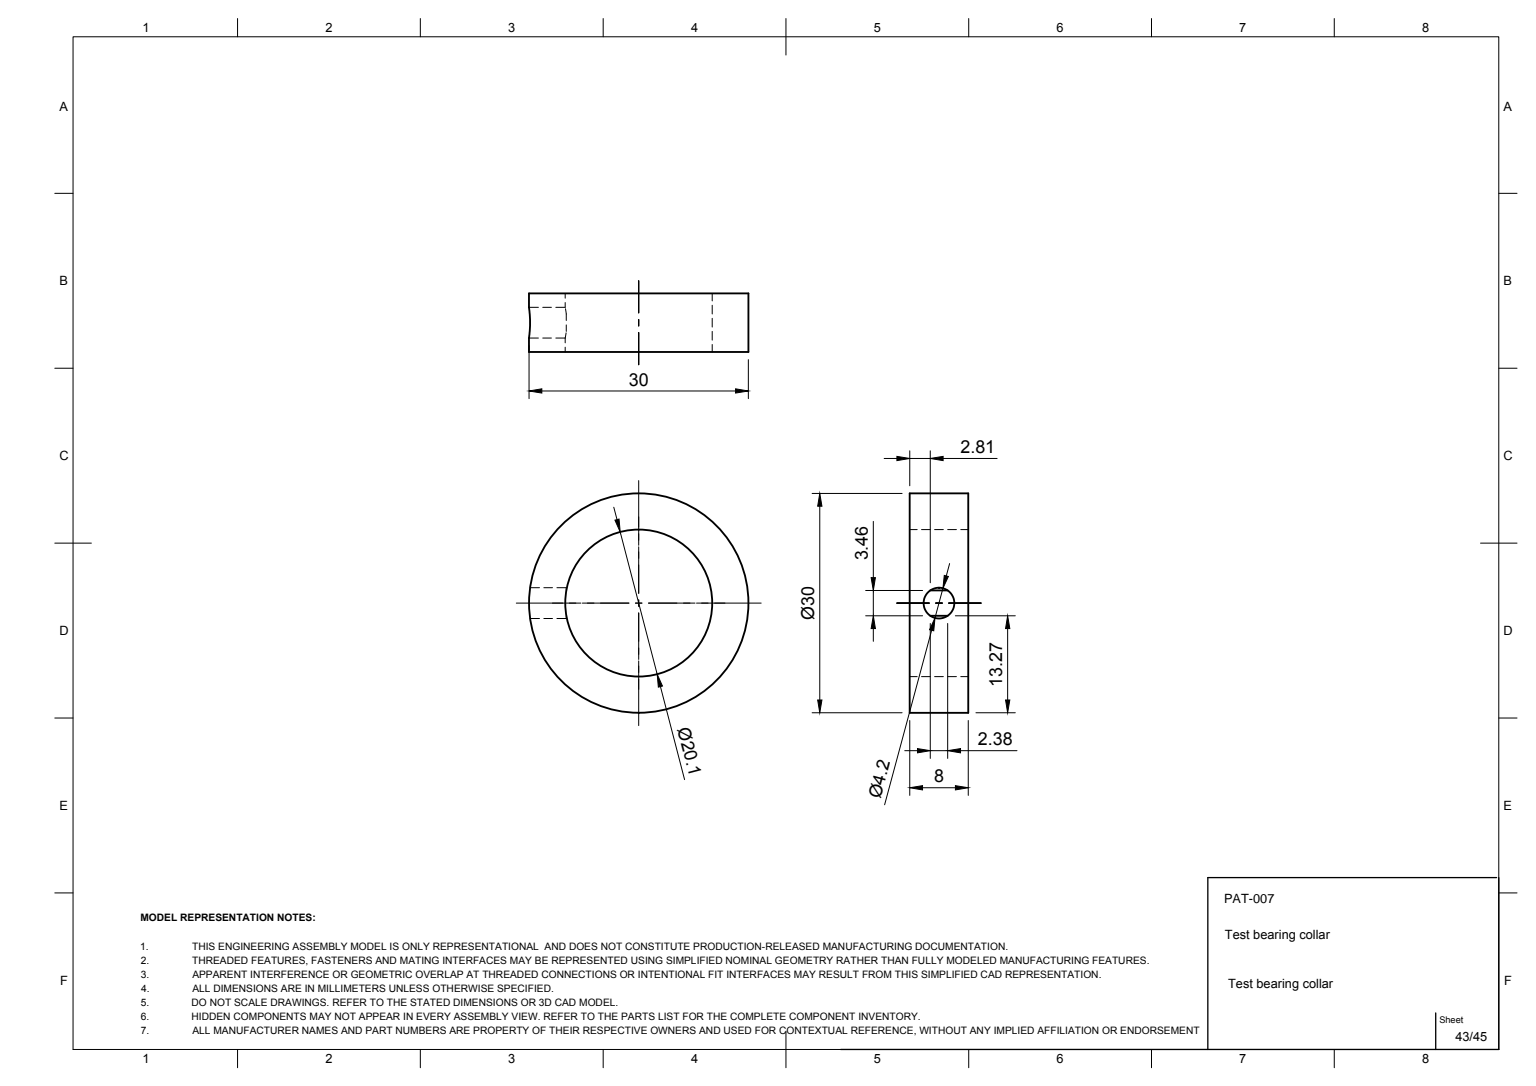
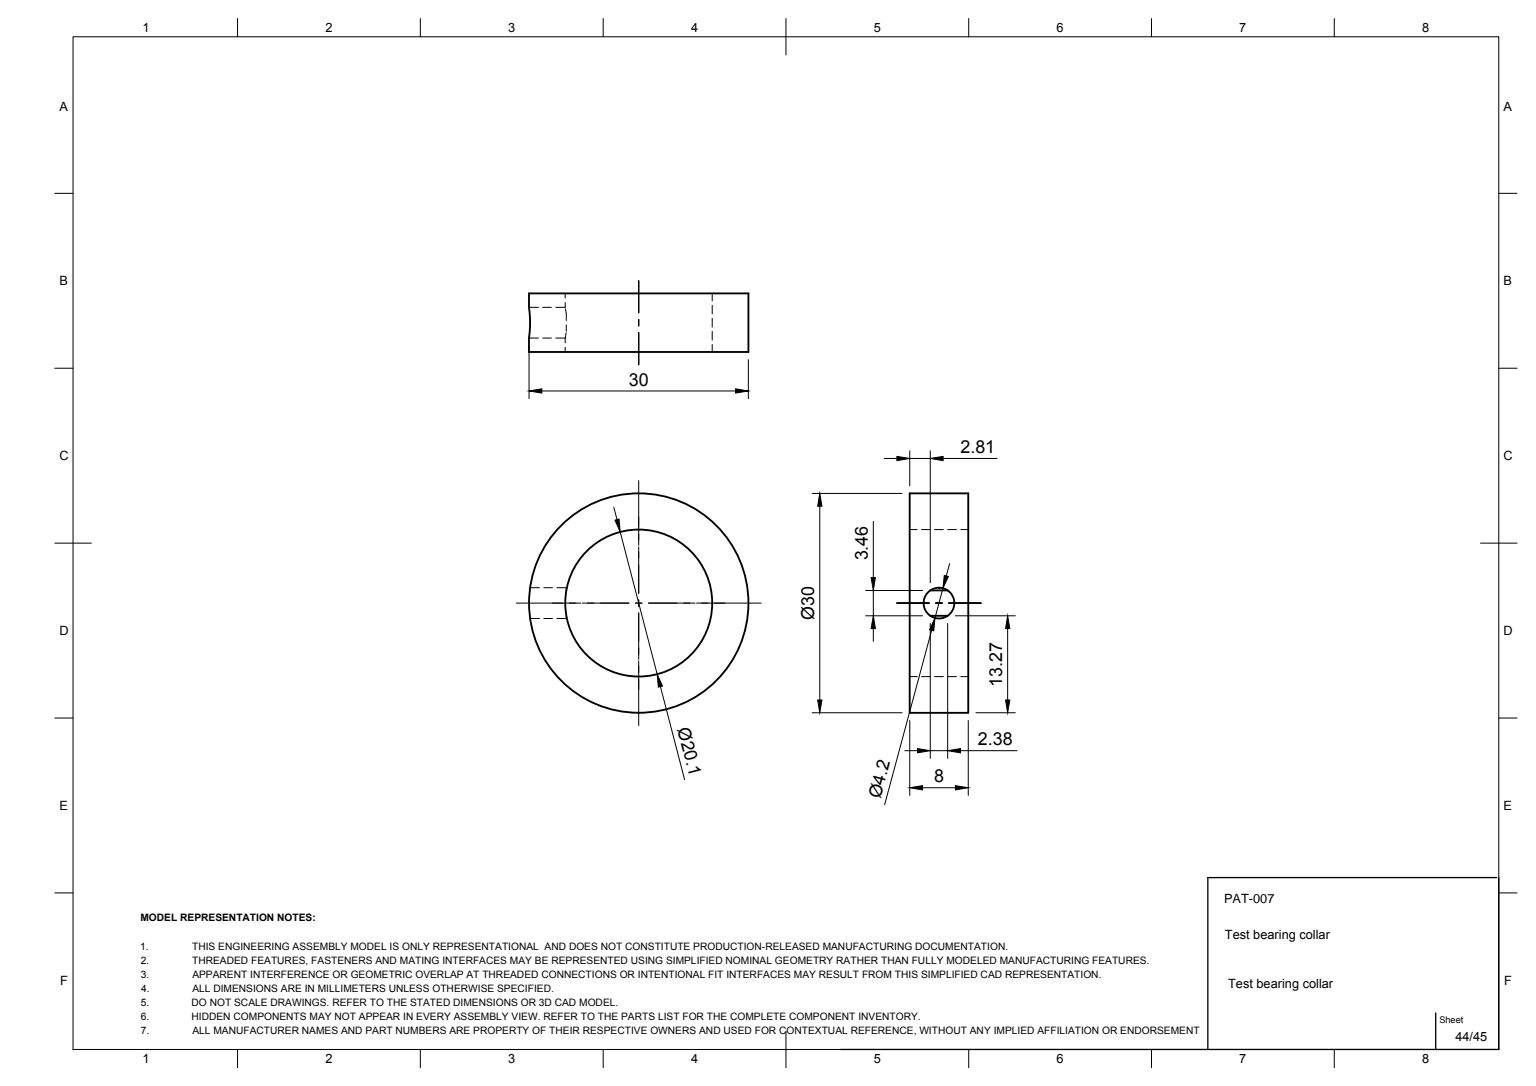
ISO-10303-21;
HEADER;
/* Generated by software containing ST-Developer
 * from STEP Tools, Inc. (www.steptools.com) 
 */

FILE_DESCRIPTION(
/* description */ ('Bearing friction torque test rig'),
/* implementation_level */ '2;1');

FILE_NAME(
/* name */ 'Test bearing collar.step',
/* time_stamp */ '2026-10-28T03:24:04-07:00',
/* author */ (''),
/* organization */ (''),
/* preprocessor_version */ 'ST-DEVELOPER v20.2',
/* originating_system */ 'Autodesk Translation Framework v15.17.0.0',
/* authorisation */ '');

FILE_SCHEMA (('AUTOMOTIVE_DESIGN { 1 0 10303 214 3 1 1 }'));
ENDSEC;

DATA;
#10=MECHANICAL_DESIGN_GEOMETRIC_PRESENTATION_REPRESENTATION('',(#589),#14822);
#383=B_SPLINE_CURVE_WITH_KNOTS('',3,(#14362,#14363,#14364,#14365,#14366,
#14367,#14368,#14369,#14370,#14371,#14372,#14373,#14374,#14375),
 .UNSPECIFIED.,.F.,.F.,(4,2,2,2,2,2,4),(0.75600573798702,0.793568827564647,
0.872922520054202,0.952276212543757,1.03162990503331,1.11098359752287,1.14854668710049),
 .UNSPECIFIED.);
#384=B_SPLINE_CURVE_WITH_KNOTS('',3,(#14381,#14382,#14383,#14384,#14385,
#14386,#14387,#14388,#14389,#14390,#14391,#14392,#14393,#14394,#14395,#14396,
#14397,#14398),.UNSPECIFIED.,.F.,.F.,(4,2,2,2,2,2,2,2,4),(0.,0.079216580773363,
0.158433161546726,0.23764869707457,0.316864232602414,0.396079768130259,
0.475295303658103,0.554511884431466,0.633728465204829),.UNSPECIFIED.);
#385=B_SPLINE_CURVE_WITH_KNOTS('',3,(#14399,#14400,#14401,#14402,#14403,
#14404,#14405,#14406,#14407,#14408,#14409,#14410,#14411,#14412,#14413,#14414,
#14415,#14416),.UNSPECIFIED.,.F.,.F.,(4,2,2,2,2,2,2,2,4),(0.633728465204829,
0.712945045978192,0.792161626751555,0.871377162279399,0.950592697807243,
1.02980823333509,1.10902376886293,1.18824034963629,1.26745693040966),
 .UNSPECIFIED.);
#386=B_SPLINE_CURVE_WITH_KNOTS('',3,(#14419,#14420,#14421,#14422,#14423,
#14424,#14425,#14426,#14427,#14428,#14429,#14430,#14431,#14432),
 .UNSPECIFIED.,.F.,.F.,(4,2,2,2,2,2,4),(0.121154929624515,0.158718019202143,
0.238071711691697,0.317425404181252,0.396779096670807,0.476132789160362,
0.513695878737989),.UNSPECIFIED.);
#496=SHAPE_REPRESENTATION_RELATIONSHIP('SRR','None',#15038,#535);
#535=ADVANCED_BREP_SHAPE_REPRESENTATION('',(#640),#14818);
#589=STYLED_ITEM('',(#15284),#640);
#640=MANIFOLD_SOLID_BREP('Body1',#7708);
#852=FACE_BOUND('',#2162,.T.);
#853=FACE_BOUND('',#2164,.T.);
#854=FACE_BOUND('',#2166,.T.);
#855=FACE_BOUND('',#2168,.T.);
#1077=PLANE('',#9072);
#1078=PLANE('',#9077);
#1079=PLANE('',#9084);
#1080=PLANE('',#9085);
#1505=FACE_OUTER_BOUND('',#2158,.T.);
#1506=FACE_OUTER_BOUND('',#2159,.T.);
#1507=FACE_OUTER_BOUND('',#2160,.T.);
#1508=FACE_OUTER_BOUND('',#2161,.T.);
#1509=FACE_OUTER_BOUND('',#2163,.T.);
#1510=FACE_OUTER_BOUND('',#2165,.T.);
#1511=FACE_OUTER_BOUND('',#2167,.T.);
#2158=EDGE_LOOP('',(#6868,#6869));
#2159=EDGE_LOOP('',(#6870,#6871,#6872,#6873,#6874,#6875,#6876,#6877,#6878));
#2160=EDGE_LOOP('',(#6879,#6880,#6881));
#2161=EDGE_LOOP('',(#6882,#6883,#6884,#6885));
#2162=EDGE_LOOP('',(#6886,#6887,#6888,#6889));
#2163=EDGE_LOOP('',(#6890,#6891,#6892,#6893));
#2164=EDGE_LOOP('',(#6894,#6895));
#2165=EDGE_LOOP('',(#6896));
#2166=EDGE_LOOP('',(#6897));
#2167=EDGE_LOOP('',(#6898));
#2168=EDGE_LOOP('',(#6899));
#2622=LINE('',#14358,#3066);
#2623=LINE('',#14379,#3067);
#2624=LINE('',#14434,#3068);
#2625=LINE('',#14439,#3069);
#2626=LINE('',#14445,#3070);
#3066=VECTOR('',#11431,1.);
#3067=VECTOR('',#11438,0.21);
#3068=VECTOR('',#11443,1.);
#3069=VECTOR('',#11448,1.005);
#3070=VECTOR('',#11455,1.5);
#3518=CIRCLE('',#9073,0.21);
#3519=CIRCLE('',#9075,0.21);
#3520=CIRCLE('',#9076,0.21);
#3521=CIRCLE('',#9079,1.005);
#3522=CIRCLE('',#9080,1.005);
#3523=CIRCLE('',#9082,1.5);
#3524=CIRCLE('',#9083,1.5);
#4141=VERTEX_POINT('',#14356);
#4142=VERTEX_POINT('',#14357);
#4143=VERTEX_POINT('',#14361);
#4144=VERTEX_POINT('',#14376);
#4145=VERTEX_POINT('',#14378);
#4146=VERTEX_POINT('',#14380);
#4147=VERTEX_POINT('',#14417);
#4148=VERTEX_POINT('',#14436);
#4149=VERTEX_POINT('',#14438);
#4150=VERTEX_POINT('',#14442);
#4151=VERTEX_POINT('',#14444);
#5060=EDGE_CURVE('',#4141,#4142,#2622,.T.);
#5061=EDGE_CURVE('',#4141,#4142,#3518,.T.);
#5062=EDGE_CURVE('',#4143,#4141,#383,.T.);
#5063=EDGE_CURVE('',#4144,#4143,#3519,.T.);
#5064=EDGE_CURVE('',#4144,#4145,#2623,.T.);
#5065=EDGE_CURVE('',#4146,#4145,#384,.T.);
#5066=EDGE_CURVE('',#4145,#4146,#385,.T.);
#5067=EDGE_CURVE('',#4147,#4144,#3520,.T.);
#5068=EDGE_CURVE('',#4142,#4147,#386,.T.);
#5069=EDGE_CURVE('',#4147,#4143,#2624,.T.);
#5070=EDGE_CURVE('',#4148,#4148,#3521,.T.);
#5071=EDGE_CURVE('',#4148,#4149,#2625,.T.);
#5072=EDGE_CURVE('',#4149,#4149,#3522,.T.);
#5073=EDGE_CURVE('',#4150,#4150,#3523,.T.);
#5074=EDGE_CURVE('',#4150,#4151,#2626,.T.);
#5075=EDGE_CURVE('',#4151,#4151,#3524,.T.);
#6868=ORIENTED_EDGE('',*,*,#5060,.F.);
#6869=ORIENTED_EDGE('',*,*,#5061,.T.);
#6870=ORIENTED_EDGE('',*,*,#5062,.F.);
#6871=ORIENTED_EDGE('',*,*,#5063,.F.);
#6872=ORIENTED_EDGE('',*,*,#5064,.T.);
#6873=ORIENTED_EDGE('',*,*,#5065,.F.);
#6874=ORIENTED_EDGE('',*,*,#5066,.F.);
#6875=ORIENTED_EDGE('',*,*,#5064,.F.);
#6876=ORIENTED_EDGE('',*,*,#5067,.F.);
#6877=ORIENTED_EDGE('',*,*,#5068,.F.);
#6878=ORIENTED_EDGE('',*,*,#5061,.F.);
#6879=ORIENTED_EDGE('',*,*,#5069,.F.);
#6880=ORIENTED_EDGE('',*,*,#5067,.T.);
#6881=ORIENTED_EDGE('',*,*,#5063,.T.);
#6882=ORIENTED_EDGE('',*,*,#5070,.F.);
#6883=ORIENTED_EDGE('',*,*,#5071,.T.);
#6884=ORIENTED_EDGE('',*,*,#5072,.T.);
#6885=ORIENTED_EDGE('',*,*,#5071,.F.);
#6886=ORIENTED_EDGE('',*,*,#5068,.T.);
#6887=ORIENTED_EDGE('',*,*,#5069,.T.);
#6888=ORIENTED_EDGE('',*,*,#5062,.T.);
#6889=ORIENTED_EDGE('',*,*,#5060,.T.);
#6890=ORIENTED_EDGE('',*,*,#5073,.F.);
#6891=ORIENTED_EDGE('',*,*,#5074,.T.);
#6892=ORIENTED_EDGE('',*,*,#5075,.T.);
#6893=ORIENTED_EDGE('',*,*,#5074,.F.);
#6894=ORIENTED_EDGE('',*,*,#5065,.T.);
#6895=ORIENTED_EDGE('',*,*,#5066,.T.);
#6896=ORIENTED_EDGE('',*,*,#5073,.T.);
#6897=ORIENTED_EDGE('',*,*,#5070,.T.);
#6898=ORIENTED_EDGE('',*,*,#5075,.F.);
#6899=ORIENTED_EDGE('',*,*,#5072,.F.);
#7195=CYLINDRICAL_SURFACE('',#9074,0.21);
#7196=CYLINDRICAL_SURFACE('',#9078,1.005);
#7197=CYLINDRICAL_SURFACE('',#9081,1.5);
#7616=ADVANCED_FACE('',(#1505),#1077,.T.);
#7617=ADVANCED_FACE('',(#1506),#7195,.F.);
#7618=ADVANCED_FACE('',(#1507),#1078,.T.);
#7619=ADVANCED_FACE('',(#1508,#852),#7196,.F.);
#7620=ADVANCED_FACE('',(#1509,#853),#7197,.T.);
#7621=ADVANCED_FACE('',(#1510,#854),#1079,.T.);
#7622=ADVANCED_FACE('',(#1511,#855),#1080,.F.);
#7708=CLOSED_SHELL('',(#7616,#7617,#7618,#7619,#7620,#7621,#7622));
#9071=AXIS2_PLACEMENT_3D('',#14354,#11427,#11428);
#9072=AXIS2_PLACEMENT_3D('',#14355,#11429,#11430);
#9073=AXIS2_PLACEMENT_3D('',#14359,#11432,#11433);
#9074=AXIS2_PLACEMENT_3D('',#14360,#11434,#11435);
#9075=AXIS2_PLACEMENT_3D('',#14377,#11436,#11437);
#9076=AXIS2_PLACEMENT_3D('',#14418,#11439,#11440);
#9077=AXIS2_PLACEMENT_3D('',#14433,#11441,#11442);
#9078=AXIS2_PLACEMENT_3D('',#14435,#11444,#11445);
#9079=AXIS2_PLACEMENT_3D('',#14437,#11446,#11447);
#9080=AXIS2_PLACEMENT_3D('',#14440,#11449,#11450);
#9081=AXIS2_PLACEMENT_3D('',#14441,#11451,#11452);
#9082=AXIS2_PLACEMENT_3D('',#14443,#11453,#11454);
#9083=AXIS2_PLACEMENT_3D('',#14446,#11456,#11457);
#9084=AXIS2_PLACEMENT_3D('',#14447,#11458,#11459);
#9085=AXIS2_PLACEMENT_3D('',#14448,#11460,#11461);
#11427=DIRECTION('axis',(0.,0.,1.));
#11428=DIRECTION('refdir',(1.,0.,0.));
#11429=DIRECTION('center_axis',(0.,0.,1.));
#11430=DIRECTION('ref_axis',(1.,0.,0.));
#11431=DIRECTION('',(0.,1.,0.));
#11432=DIRECTION('center_axis',(0.,0.,1.));
#11433=DIRECTION('ref_axis',(1.,0.,0.));
#11434=DIRECTION('center_axis',(0.,0.,1.));
#11435=DIRECTION('ref_axis',(1.,0.,0.));
#11436=DIRECTION('center_axis',(0.,0.,1.));
#11437=DIRECTION('ref_axis',(1.,0.,0.));
#11438=DIRECTION('',(0.,0.,1.));
#11439=DIRECTION('center_axis',(0.,0.,1.));
#11440=DIRECTION('ref_axis',(1.,0.,0.));
#11441=DIRECTION('center_axis',(0.,0.,1.));
#11442=DIRECTION('ref_axis',(1.,0.,0.));
#11443=DIRECTION('',(0.,-1.,0.));
#11444=DIRECTION('center_axis',(0.,1.,0.));
#11445=DIRECTION('ref_axis',(1.,0.,0.));
#11446=DIRECTION('center_axis',(0.,-1.,0.));
#11447=DIRECTION('ref_axis',(1.,0.,0.));
#11448=DIRECTION('',(0.,-1.,0.));
#11449=DIRECTION('center_axis',(0.,-1.,0.));
#11450=DIRECTION('ref_axis',(1.,0.,0.));
#11451=DIRECTION('center_axis',(0.,1.,0.));
#11452=DIRECTION('ref_axis',(1.,0.,0.));
#11453=DIRECTION('center_axis',(0.,1.,0.));
#11454=DIRECTION('ref_axis',(1.,0.,0.));
#11455=DIRECTION('',(0.,-1.,0.));
#11456=DIRECTION('center_axis',(0.,1.,0.));
#11457=DIRECTION('ref_axis',(1.,0.,0.));
#11458=DIRECTION('center_axis',(0.,1.,0.));
#11459=DIRECTION('ref_axis',(1.,0.,0.));
#11460=DIRECTION('center_axis',(0.,1.,0.));
#11461=DIRECTION('ref_axis',(1.,0.,0.));
#14354=CARTESIAN_POINT('',(0.,0.,0.));
#14355=CARTESIAN_POINT('Origin',(0.,-1.1,7.99));
#14356=CARTESIAN_POINT('',(0.172988438920056,-1.21905880899792,7.99));
#14357=CARTESIAN_POINT('',(0.172988438920056,-0.980941191002085,7.99));
#14358=CARTESIAN_POINT('',(0.172988438920056,-1.5,7.99));
#14359=CARTESIAN_POINT('Origin',(0.,-1.1,7.99));
#14360=CARTESIAN_POINT('Origin',(0.,-1.1,7.99));
#14361=CARTESIAN_POINT('',(-0.172988438920056,-1.21905880899792,7.99));
#14362=CARTESIAN_POINT('Ctrl Pts',(-0.172988438920056,-1.21905880899792,
7.99));
#14363=CARTESIAN_POINT('Ctrl Pts',(-0.165594865311315,-1.22980142239529,
7.99129192197638));
#14364=CARTESIAN_POINT('Ctrl Pts',(-0.157297138725606,-1.23968770937274,
7.99265394943905));
#14365=CARTESIAN_POINT('Ctrl Pts',(-0.129892073845076,-1.26709277425327,
7.9967480843909));
#14366=CARTESIAN_POINT('Ctrl Pts',(-0.106330167759285,-1.28324205633295,
7.99969589327638));
#14367=CARTESIAN_POINT('Ctrl Pts',(-0.0546129046324105,-1.30469779396491,
8.00385029472357));
#14368=CARTESIAN_POINT('Ctrl Pts',(-0.0264512308298516,-1.31,8.005));
#14369=CARTESIAN_POINT('Ctrl Pts',(0.0264512308298515,-1.31,8.005));
#14370=CARTESIAN_POINT('Ctrl Pts',(0.0546129046324104,-1.30469779396491,
8.00385029472357));
#14371=CARTESIAN_POINT('Ctrl Pts',(0.106330167759284,-1.28324205633295,
7.99969589327638));
#14372=CARTESIAN_POINT('Ctrl Pts',(0.129892073845076,-1.26709277425327,
7.9967480843909));
#14373=CARTESIAN_POINT('Ctrl Pts',(0.157297138725606,-1.23968770937274,
7.99265394943905));
#14374=CARTESIAN_POINT('Ctrl Pts',(0.165594865311314,-1.22980142239529,
7.99129192197638));
#14375=CARTESIAN_POINT('Ctrl Pts',(0.172988438920056,-1.21905880899792,
7.99));
#14376=CARTESIAN_POINT('',(-0.21,-1.1,7.99));
#14377=CARTESIAN_POINT('Origin',(0.,-1.1,7.99));
#14378=CARTESIAN_POINT('',(-0.21,-1.1,8.48522725533839));
#14379=CARTESIAN_POINT('',(-0.21,-1.1,7.99));
#14380=CARTESIAN_POINT('',(0.21,-1.1,8.48522725533839));
#14381=CARTESIAN_POINT('Ctrl Pts',(0.21,-1.1,8.48522725533839));
#14382=CARTESIAN_POINT('Ctrl Pts',(0.21,-1.12640552692445,8.48522725533839));
#14383=CARTESIAN_POINT('Ctrl Pts',(0.204715737269596,-1.15454707409071,
8.48600415954412));
#14384=CARTESIAN_POINT('Ctrl Pts',(0.183273763036331,-1.20627626890513,
8.48880073282317));
#14385=CARTESIAN_POINT('Ctrl Pts',(0.167117923970394,-1.22986692412796,
8.49077897157582));
#14386=CARTESIAN_POINT('Ctrl Pts',(0.129867169887369,-1.26711767821098,
8.49448481141327));
#14387=CARTESIAN_POINT('Ctrl Pts',(0.106276408305765,-1.28327371000135,
8.49645455657129));
#14388=CARTESIAN_POINT('Ctrl Pts',(0.0545468514059002,-1.30471582482622,
8.49923165515646));
#14389=CARTESIAN_POINT('Ctrl Pts',(0.0264051785092814,-1.31,8.5));
#14390=CARTESIAN_POINT('Ctrl Pts',(-0.0264051785092814,-1.31,8.5));
#14391=CARTESIAN_POINT('Ctrl Pts',(-0.0545468514059001,-1.30471582482622,
8.49923165515646));
#14392=CARTESIAN_POINT('Ctrl Pts',(-0.106276408305765,-1.28327371000135,
8.49645455657129));
#14393=CARTESIAN_POINT('Ctrl Pts',(-0.129867169887369,-1.26711767821098,
8.49448481141327));
#14394=CARTESIAN_POINT('Ctrl Pts',(-0.167117923970394,-1.22986692412796,
8.49077897157582));
#14395=CARTESIAN_POINT('Ctrl Pts',(-0.183273763036331,-1.20627626890513,
8.48880073282317));
#14396=CARTESIAN_POINT('Ctrl Pts',(-0.204715737269596,-1.15454707409071,
8.48600415954412));
#14397=CARTESIAN_POINT('Ctrl Pts',(-0.21,-1.12640552692445,8.48522725533839));
#14398=CARTESIAN_POINT('Ctrl Pts',(-0.21,-1.1,8.48522725533839));
#14399=CARTESIAN_POINT('Ctrl Pts',(-0.21,-1.1,8.48522725533839));
#14400=CARTESIAN_POINT('Ctrl Pts',(-0.21,-1.07359447307555,8.48522725533839));
#14401=CARTESIAN_POINT('Ctrl Pts',(-0.204715737269596,-1.04545292590929,
8.48600415954412));
#14402=CARTESIAN_POINT('Ctrl Pts',(-0.183273763036331,-0.993723731094873,
8.48880073282317));
#14403=CARTESIAN_POINT('Ctrl Pts',(-0.167117923970394,-0.970133075872044,
8.49077897157582));
#14404=CARTESIAN_POINT('Ctrl Pts',(-0.129867169887369,-0.932882321789019,
8.49448481141327));
#14405=CARTESIAN_POINT('Ctrl Pts',(-0.106276408305765,-0.916726289998648,
8.49645455657129));
#14406=CARTESIAN_POINT('Ctrl Pts',(-0.0545468514059001,-0.895284175173782,
8.49923165515646));
#14407=CARTESIAN_POINT('Ctrl Pts',(-0.0264051785092814,-0.89,8.5));
#14408=CARTESIAN_POINT('Ctrl Pts',(0.0264051785092814,-0.89,8.5));
#14409=CARTESIAN_POINT('Ctrl Pts',(0.0545468514059001,-0.895284175173782,
8.49923165515645));
#14410=CARTESIAN_POINT('Ctrl Pts',(0.106276408305765,-0.916726289998648,
8.49645455657129));
#14411=CARTESIAN_POINT('Ctrl Pts',(0.129867169887369,-0.932882321789019,
8.49448481141327));
#14412=CARTESIAN_POINT('Ctrl Pts',(0.167117923970394,-0.970133075872044,
8.49077897157582));
#14413=CARTESIAN_POINT('Ctrl Pts',(0.183273763036331,-0.993723731094873,
8.48880073282317));
#14414=CARTESIAN_POINT('Ctrl Pts',(0.204715737269596,-1.04545292590929,
8.48600415954412));
#14415=CARTESIAN_POINT('Ctrl Pts',(0.21,-1.07359447307555,8.48522725533839));
#14416=CARTESIAN_POINT('Ctrl Pts',(0.21,-1.1,8.48522725533839));
#14417=CARTESIAN_POINT('',(-0.172988438920056,-0.980941191002085,7.99));
#14418=CARTESIAN_POINT('Origin',(0.,-1.1,7.99));
#14419=CARTESIAN_POINT('Ctrl Pts',(0.172988438920056,-0.980941191002085,
7.99));
#14420=CARTESIAN_POINT('Ctrl Pts',(0.165594865311315,-0.970198577604708,
7.99129192197638));
#14421=CARTESIAN_POINT('Ctrl Pts',(0.157297138725606,-0.960312290627256,
7.99265394943905));
#14422=CARTESIAN_POINT('Ctrl Pts',(0.129892073845076,-0.932907225746726,
7.9967480843909));
#14423=CARTESIAN_POINT('Ctrl Pts',(0.106330167759284,-0.916757943667051,
7.99969589327638));
#14424=CARTESIAN_POINT('Ctrl Pts',(0.0546129046324105,-0.895302206035094,
8.00385029472357));
#14425=CARTESIAN_POINT('Ctrl Pts',(0.0264512308298516,-0.89,8.005));
#14426=CARTESIAN_POINT('Ctrl Pts',(-0.0264512308298516,-0.89,8.005));
#14427=CARTESIAN_POINT('Ctrl Pts',(-0.0546129046324105,-0.895302206035094,
8.00385029472357));
#14428=CARTESIAN_POINT('Ctrl Pts',(-0.106330167759284,-0.916757943667051,
7.99969589327638));
#14429=CARTESIAN_POINT('Ctrl Pts',(-0.129892073845076,-0.932907225746726,
7.9967480843909));
#14430=CARTESIAN_POINT('Ctrl Pts',(-0.157297138725606,-0.960312290627256,
7.99265394943905));
#14431=CARTESIAN_POINT('Ctrl Pts',(-0.165594865311314,-0.970198577604708,
7.99129192197638));
#14432=CARTESIAN_POINT('Ctrl Pts',(-0.172988438920056,-0.980941191002085,
7.99));
#14433=CARTESIAN_POINT('Origin',(0.,-1.1,7.99));
#14434=CARTESIAN_POINT('',(-0.172988438920056,-1.5,7.99));
#14435=CARTESIAN_POINT('Origin',(0.,-1.5,7.));
#14436=CARTESIAN_POINT('',(-1.005,-0.7,7.));
#14437=CARTESIAN_POINT('Origin',(0.,-0.7,7.));
#14438=CARTESIAN_POINT('',(-1.005,-1.5,7.));
#14439=CARTESIAN_POINT('',(-1.005,-1.5,7.));
#14440=CARTESIAN_POINT('Origin',(0.,-1.5,7.));
#14441=CARTESIAN_POINT('Origin',(0.,-1.5,7.));
#14442=CARTESIAN_POINT('',(-1.5,-0.7,7.));
#14443=CARTESIAN_POINT('Origin',(0.,-0.7,7.));
#14444=CARTESIAN_POINT('',(-1.5,-1.5,7.));
#14445=CARTESIAN_POINT('',(-1.5,-1.5,7.));
#14446=CARTESIAN_POINT('Origin',(0.,-1.5,7.));
#14447=CARTESIAN_POINT('Origin',(0.,-0.7,7.));
#14448=CARTESIAN_POINT('Origin',(0.,-1.5,7.));
#14773=UNCERTAINTY_MEASURE_WITH_UNIT(LENGTH_MEASURE(0.001),#14823,
'DISTANCE_ACCURACY_VALUE',
'Maximum model space distance between geometric entities at asserted c
onnectivities');
#14777=UNCERTAINTY_MEASURE_WITH_UNIT(LENGTH_MEASURE(0.001),#14823,
'DISTANCE_ACCURACY_VALUE',
'Maximum model space distance between geometric entities at asserted c
onnectivities');
#14818=(
GEOMETRIC_REPRESENTATION_CONTEXT(3)
GLOBAL_UNCERTAINTY_ASSIGNED_CONTEXT((#14773))
GLOBAL_UNIT_ASSIGNED_CONTEXT((#14823,#14825,#14826))
REPRESENTATION_CONTEXT('','3D')
);
#14822=(
GEOMETRIC_REPRESENTATION_CONTEXT(3)
GLOBAL_UNCERTAINTY_ASSIGNED_CONTEXT((#14777))
GLOBAL_UNIT_ASSIGNED_CONTEXT((#14823,#14825,#14826))
REPRESENTATION_CONTEXT('','3D')
);
#14823=(
LENGTH_UNIT()
NAMED_UNIT(*)
SI_UNIT(.CENTI.,.METRE.)
);
#14825=(
NAMED_UNIT(*)
PLANE_ANGLE_UNIT()
SI_UNIT($,.RADIAN.)
);
#14826=(
NAMED_UNIT(*)
SI_UNIT($,.STERADIAN.)
SOLID_ANGLE_UNIT()
);
#14867=SHAPE_DEFINITION_REPRESENTATION(#14977,#15038);
#14977=PRODUCT_DEFINITION_SHAPE('',$,#15083);
#15038=SHAPE_REPRESENTATION('',(#9071),#14818);
#15042=PRODUCT_DEFINITION_CONTEXT('part definition',#15176,'design');
#15083=PRODUCT_DEFINITION('Test bearing collar','Test bearing collar',#15127,
#15042);
#15127=PRODUCT_DEFINITION_FORMATION('',$,#15218);
#15176=APPLICATION_CONTEXT(
'Core Data for Automotive Mechanical Design Process');
#15177=PRODUCT_CONTEXT('part definition',#15176,'mechanical');
#15218=PRODUCT('Test bearing collar','Test bearing collar',
'Test bearing collar',(#15177));
#15278=COLOUR_RGB('Grey',0.48,0.52,0.57);
#15279=FILL_AREA_STYLE_COLOUR('',#15278);
#15280=FILL_AREA_STYLE('',(#15279));
#15281=SURFACE_STYLE_FILL_AREA(#15280);
#15282=SURFACE_SIDE_STYLE('',(#15281));
#15283=SURFACE_STYLE_USAGE(.BOTH.,#15282);
#15284=PRESENTATION_STYLE_ASSIGNMENT((#15283));
ENDSEC;
END-ISO-10303-21;
